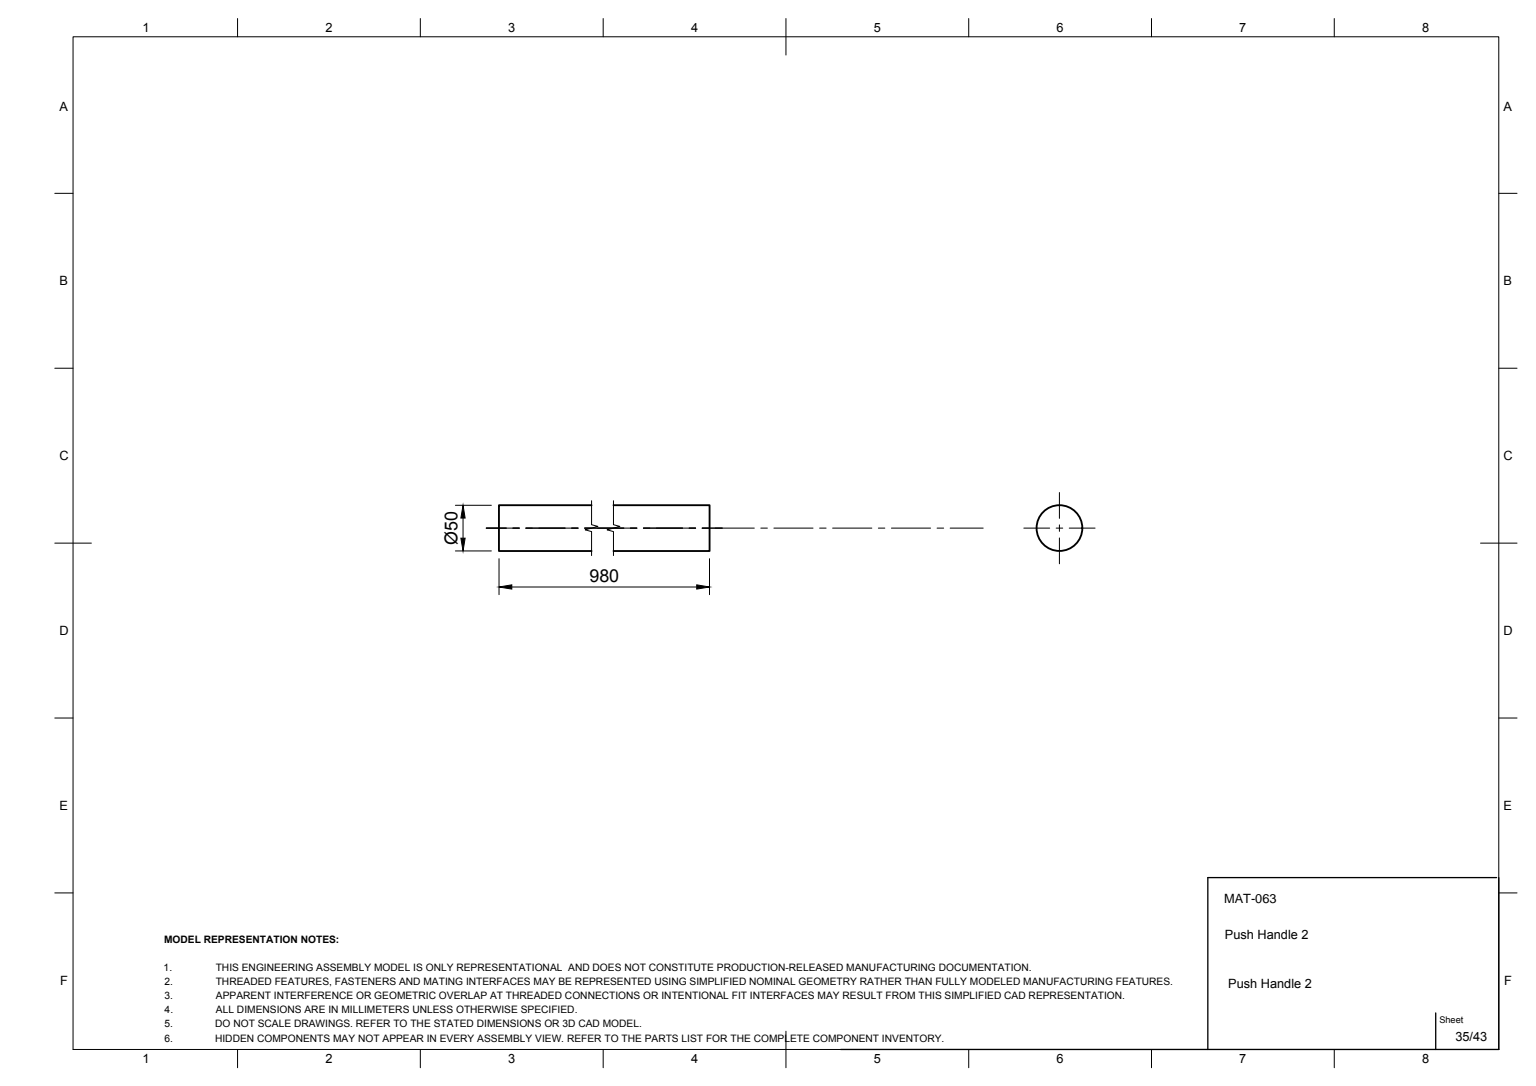
ISO-10303-21;
HEADER;
/* Generated by software containing ST-Developer
 * from STEP Tools, Inc. (www.steptools.com) 
 */

FILE_DESCRIPTION(
/* description */ (''),
/* implementation_level */ '2;1');

FILE_NAME(
/* name */ 'Push Handle 2.step',
/* time_stamp */ '2026-10-24T09:43:01-07:00',
/* author */ (''),
/* organization */ (''),
/* preprocessor_version */ 'ST-DEVELOPER v20.2',
/* originating_system */ 'Autodesk Translation Framework v15.15.0.0',
/* authorisation */ '');

FILE_SCHEMA (('AUTOMOTIVE_DESIGN { 1 0 10303 214 3 1 1 }'));
ENDSEC;

DATA;
#10=MECHANICAL_DESIGN_GEOMETRIC_PRESENTATION_REPRESENTATION('',(#298),#11112);
#232=SHAPE_REPRESENTATION_RELATIONSHIP('SRR','None',#11258,#265);
#265=ADVANCED_BREP_SHAPE_REPRESENTATION('',(#331),#11103);
#298=STYLED_ITEM('',(#11426),#331);
#331=MANIFOLD_SOLID_BREP('Push Handle 2',#6035);
#648=PLANE('',#7156);
#649=PLANE('',#7157);
#1000=FACE_OUTER_BOUND('',#1504,.T.);
#1001=FACE_OUTER_BOUND('',#1505,.T.);
#1002=FACE_OUTER_BOUND('',#1506,.T.);
#1504=EDGE_LOOP('',(#5375,#5376,#5377,#5378));
#1505=EDGE_LOOP('',(#5379));
#1506=EDGE_LOOP('',(#5380));
#1893=LINE('',#10866,#2252);
#2252=VECTOR('',#9091,0.025);
#2648=CIRCLE('',#7154,0.025);
#2649=CIRCLE('',#7155,0.025);
#3138=VERTEX_POINT('',#10863);
#3139=VERTEX_POINT('',#10865);
#3891=EDGE_CURVE('',#3138,#3138,#2648,.F.);
#3892=EDGE_CURVE('',#3138,#3139,#1893,.T.);
#3893=EDGE_CURVE('',#3139,#3139,#2649,.T.);
#5375=ORIENTED_EDGE('',*,*,#3891,.T.);
#5376=ORIENTED_EDGE('',*,*,#3892,.T.);
#5377=ORIENTED_EDGE('',*,*,#3893,.T.);
#5378=ORIENTED_EDGE('',*,*,#3892,.F.);
#5379=ORIENTED_EDGE('',*,*,#3893,.F.);
#5380=ORIENTED_EDGE('',*,*,#3891,.F.);
#5626=CYLINDRICAL_SURFACE('',#7153,0.025);
#5973=ADVANCED_FACE('',(#1000),#5626,.T.);
#5974=ADVANCED_FACE('',(#1001),#648,.T.);
#5975=ADVANCED_FACE('',(#1002),#649,.F.);
#6035=CLOSED_SHELL('',(#5973,#5974,#5975));
#7152=AXIS2_PLACEMENT_3D('',#10861,#9085,#9086);
#7153=AXIS2_PLACEMENT_3D('',#10862,#9087,#9088);
#7154=AXIS2_PLACEMENT_3D('',#10864,#9089,#9090);
#7155=AXIS2_PLACEMENT_3D('',#10867,#9092,#9093);
#7156=AXIS2_PLACEMENT_3D('',#10868,#9094,#9095);
#7157=AXIS2_PLACEMENT_3D('',#10869,#9096,#9097);
#9085=DIRECTION('axis',(0.,0.,1.));
#9086=DIRECTION('refdir',(1.,0.,0.));
#9087=DIRECTION('center_axis',(1.,0.,0.));
#9088=DIRECTION('ref_axis',(0.,0.,-1.));
#9089=DIRECTION('center_axis',(1.,0.,0.));
#9090=DIRECTION('ref_axis',(0.,0.,-1.));
#9091=DIRECTION('',(-1.,0.,0.));
#9092=DIRECTION('center_axis',(1.,0.,0.));
#9093=DIRECTION('ref_axis',(0.,0.,-1.));
#9094=DIRECTION('center_axis',(-1.,2.37904933965006E-16,7.4543545972162E-17));
#9095=DIRECTION('ref_axis',(-2.37904933965006E-16,-1.,1.16006348247081E-48));
#9096=DIRECTION('center_axis',(-1.,-2.37904933965006E-16,-7.4543545972162E-17));
#9097=DIRECTION('ref_axis',(2.37904933965006E-16,-1.,1.16006348247081E-48));
#10861=CARTESIAN_POINT('',(0.,0.,0.));
#10862=CARTESIAN_POINT('Origin',(-0.560710678,0.3,-0.955882353));
#10863=CARTESIAN_POINT('',(0.49,0.3,-0.930882353));
#10864=CARTESIAN_POINT('Origin',(0.49,0.3,-0.955882353));
#10865=CARTESIAN_POINT('',(-0.49,0.3,-0.930882353));
#10866=CARTESIAN_POINT('',(-0.560710678,0.3,-0.930882353));
#10867=CARTESIAN_POINT('Origin',(-0.49,0.3,-0.955882353));
#10868=CARTESIAN_POINT('Origin',(-0.49,0.3,-0.955882352999999));
#10869=CARTESIAN_POINT('Origin',(0.49,0.3,-0.955882352999999));
#11064=UNCERTAINTY_MEASURE_WITH_UNIT(LENGTH_MEASURE(1.E-5),#11113,
'DISTANCE_ACCURACY_VALUE',
'Maximum model space distance between geometric entities at asserted c
onnectivities');
#11073=UNCERTAINTY_MEASURE_WITH_UNIT(LENGTH_MEASURE(1.E-5),#11113,
'DISTANCE_ACCURACY_VALUE',
'Maximum model space distance between geometric entities at asserted c
onnectivities');
#11103=(
GEOMETRIC_REPRESENTATION_CONTEXT(3)
GLOBAL_UNCERTAINTY_ASSIGNED_CONTEXT((#11064))
GLOBAL_UNIT_ASSIGNED_CONTEXT((#11113,#11114,#11115))
REPRESENTATION_CONTEXT('','3D')
);
#11112=(
GEOMETRIC_REPRESENTATION_CONTEXT(3)
GLOBAL_UNCERTAINTY_ASSIGNED_CONTEXT((#11073))
GLOBAL_UNIT_ASSIGNED_CONTEXT((#11113,#11114,#11115))
REPRESENTATION_CONTEXT('','3D')
);
#11113=(
LENGTH_UNIT()
NAMED_UNIT(*)
SI_UNIT($,.METRE.)
);
#11114=(
NAMED_UNIT(*)
PLANE_ANGLE_UNIT()
SI_UNIT($,.RADIAN.)
);
#11115=(
NAMED_UNIT(*)
SI_UNIT($,.STERADIAN.)
SOLID_ANGLE_UNIT()
);
#11145=SHAPE_DEFINITION_REPRESENTATION(#11196,#11258);
#11196=PRODUCT_DEFINITION_SHAPE('',$,#11297);
#11258=SHAPE_REPRESENTATION('',(#7152),#11103);
#11267=PRODUCT_DEFINITION_CONTEXT('part definition',#11383,'design');
#11297=PRODUCT_DEFINITION('Push Handle 2','Push Handle 2',#11335,#11267);
#11335=PRODUCT_DEFINITION_FORMATION('',$,#11414);
#11383=APPLICATION_CONTEXT(
'Core Data for Automotive Mechanical Design Process');
#11384=PRODUCT_CONTEXT('part definition',#11383,'mechanical');
#11414=PRODUCT('Push Handle 2','Push Handle 2',
'back_push__ DE     2589',(#11384));
#11426=PRESENTATION_STYLE_ASSIGNMENT((#11430));
#11430=SURFACE_STYLE_USAGE(.BOTH.,#11434);
#11434=SURFACE_SIDE_STYLE('',(#11438));
#11438=SURFACE_STYLE_FILL_AREA(#11442);
#11442=FILL_AREA_STYLE('Opaque(202,209,238)',(#11446));
#11446=FILL_AREA_STYLE_COLOUR('Opaque(202,209,238)',#11450);
#11450=COLOUR_RGB('Opaque(202,209,238)',0.792156862745098,0.819607843137255,
0.933333333333333);
ENDSEC;
END-ISO-10303-21;
